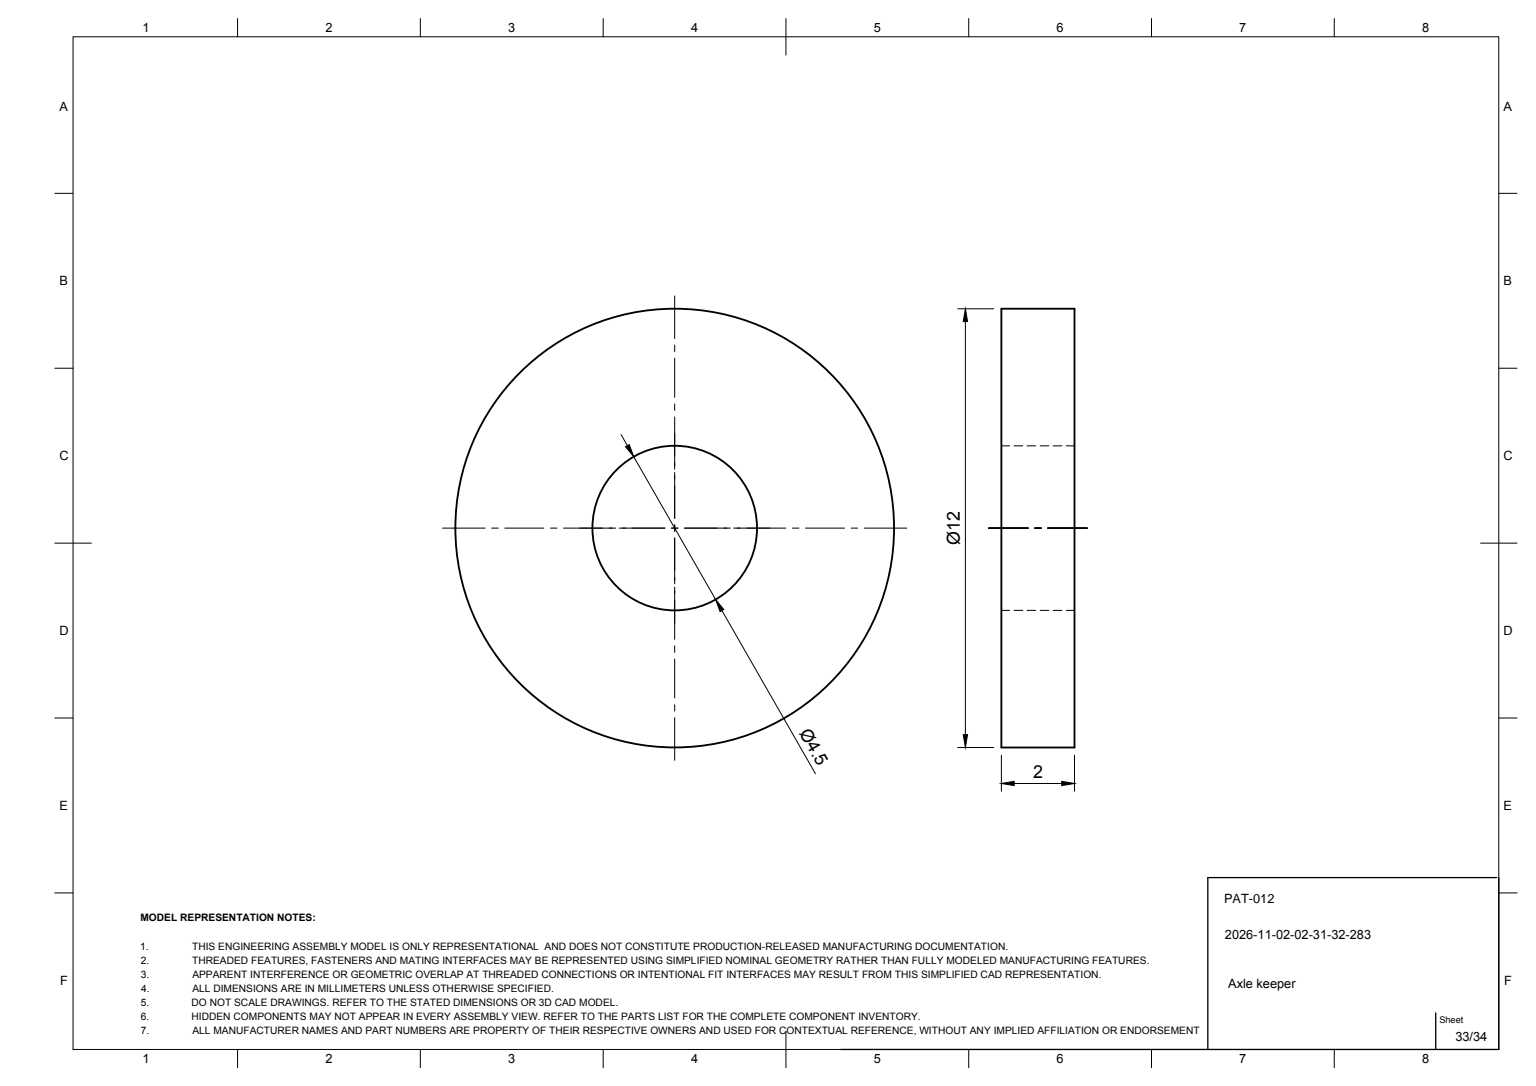
ISO-10303-21;
HEADER;
/* Generated by software containing ST-Developer
 * from STEP Tools, Inc. (www.steptools.com) 
 */

FILE_DESCRIPTION(
/* description */ ('Belt tensioner idler arm'),
/* implementation_level */ '2;1');

FILE_NAME(
/* name */ 'Axle keeper.step',
/* time_stamp */ '2026-10-28T03:22:15-07:00',
/* author */ (''),
/* organization */ (''),
/* preprocessor_version */ 'ST-DEVELOPER v20.2',
/* originating_system */ 'Autodesk Translation Framework v15.17.0.0',
/* authorisation */ '');

FILE_SCHEMA (('AUTOMOTIVE_DESIGN { 1 0 10303 214 3 1 1 }'));
ENDSEC;

DATA;
#10=MECHANICAL_DESIGN_GEOMETRIC_PRESENTATION_REPRESENTATION('',(#485),#12779);
#409=SHAPE_REPRESENTATION_RELATIONSHIP('SRR','None',#12958,#443);
#443=ADVANCED_BREP_SHAPE_REPRESENTATION('',(#524),#12775);
#485=STYLED_ITEM('',(#13184),#524);
#524=MANIFOLD_SOLID_BREP('Body1',#6222);
#648=FACE_BOUND('',#1611,.T.);
#649=FACE_BOUND('',#1613,.T.);
#810=PLANE('',#7218);
#811=PLANE('',#7219);
#1120=FACE_OUTER_BOUND('',#1608,.T.);
#1121=FACE_OUTER_BOUND('',#1609,.T.);
#1122=FACE_OUTER_BOUND('',#1610,.T.);
#1123=FACE_OUTER_BOUND('',#1612,.T.);
#1608=EDGE_LOOP('',(#5224,#5225,#5226,#5227));
#1609=EDGE_LOOP('',(#5228,#5229,#5230,#5231));
#1610=EDGE_LOOP('',(#5232));
#1611=EDGE_LOOP('',(#5233));
#1612=EDGE_LOOP('',(#5234));
#1613=EDGE_LOOP('',(#5235));
#1961=LINE('',#11940,#2310);
#1962=LINE('',#11946,#2311);
#2310=VECTOR('',#8911,0.225);
#2311=VECTOR('',#8918,0.6);
#2667=CIRCLE('',#7213,0.225);
#2668=CIRCLE('',#7214,0.225);
#2669=CIRCLE('',#7216,0.6);
#2670=CIRCLE('',#7217,0.6);
#3150=VERTEX_POINT('',#11937);
#3151=VERTEX_POINT('',#11939);
#3152=VERTEX_POINT('',#11943);
#3153=VERTEX_POINT('',#11945);
#3867=EDGE_CURVE('',#3150,#3150,#2667,.T.);
#3868=EDGE_CURVE('',#3150,#3151,#1961,.T.);
#3869=EDGE_CURVE('',#3151,#3151,#2668,.T.);
#3870=EDGE_CURVE('',#3152,#3152,#2669,.T.);
#3871=EDGE_CURVE('',#3152,#3153,#1962,.T.);
#3872=EDGE_CURVE('',#3153,#3153,#2670,.T.);
#5224=ORIENTED_EDGE('',*,*,#3867,.F.);
#5225=ORIENTED_EDGE('',*,*,#3868,.T.);
#5226=ORIENTED_EDGE('',*,*,#3869,.T.);
#5227=ORIENTED_EDGE('',*,*,#3868,.F.);
#5228=ORIENTED_EDGE('',*,*,#3870,.F.);
#5229=ORIENTED_EDGE('',*,*,#3871,.T.);
#5230=ORIENTED_EDGE('',*,*,#3872,.T.);
#5231=ORIENTED_EDGE('',*,*,#3871,.F.);
#5232=ORIENTED_EDGE('',*,*,#3870,.T.);
#5233=ORIENTED_EDGE('',*,*,#3867,.T.);
#5234=ORIENTED_EDGE('',*,*,#3872,.F.);
#5235=ORIENTED_EDGE('',*,*,#3869,.F.);
#5761=CYLINDRICAL_SURFACE('',#7212,0.225);
#5762=CYLINDRICAL_SURFACE('',#7215,0.6);
#6097=ADVANCED_FACE('',(#1120),#5761,.F.);
#6098=ADVANCED_FACE('',(#1121),#5762,.T.);
#6099=ADVANCED_FACE('',(#1122,#648),#810,.T.);
#6100=ADVANCED_FACE('',(#1123,#649),#811,.F.);
#6222=CLOSED_SHELL('',(#6097,#6098,#6099,#6100));
#7211=AXIS2_PLACEMENT_3D('',#11935,#8905,#8906);
#7212=AXIS2_PLACEMENT_3D('',#11936,#8907,#8908);
#7213=AXIS2_PLACEMENT_3D('',#11938,#8909,#8910);
#7214=AXIS2_PLACEMENT_3D('',#11941,#8912,#8913);
#7215=AXIS2_PLACEMENT_3D('',#11942,#8914,#8915);
#7216=AXIS2_PLACEMENT_3D('',#11944,#8916,#8917);
#7217=AXIS2_PLACEMENT_3D('',#11947,#8919,#8920);
#7218=AXIS2_PLACEMENT_3D('',#11948,#8921,#8922);
#7219=AXIS2_PLACEMENT_3D('',#11949,#8923,#8924);
#8905=DIRECTION('axis',(0.,0.,1.));
#8906=DIRECTION('refdir',(1.,0.,0.));
#8907=DIRECTION('center_axis',(0.,0.,1.));
#8908=DIRECTION('ref_axis',(1.,0.,0.));
#8909=DIRECTION('center_axis',(0.,0.,-1.));
#8910=DIRECTION('ref_axis',(1.,0.,0.));
#8911=DIRECTION('',(0.,0.,-1.));
#8912=DIRECTION('center_axis',(0.,0.,-1.));
#8913=DIRECTION('ref_axis',(1.,0.,0.));
#8914=DIRECTION('center_axis',(0.,0.,1.));
#8915=DIRECTION('ref_axis',(1.,0.,0.));
#8916=DIRECTION('center_axis',(0.,0.,1.));
#8917=DIRECTION('ref_axis',(1.,0.,0.));
#8918=DIRECTION('',(0.,0.,-1.));
#8919=DIRECTION('center_axis',(0.,0.,1.));
#8920=DIRECTION('ref_axis',(1.,0.,0.));
#8921=DIRECTION('center_axis',(0.,0.,1.));
#8922=DIRECTION('ref_axis',(1.,0.,0.));
#8923=DIRECTION('center_axis',(0.,0.,1.));
#8924=DIRECTION('ref_axis',(1.,0.,0.));
#11935=CARTESIAN_POINT('',(0.,0.,0.));
#11936=CARTESIAN_POINT('Origin',(9.,0.,9.));
#11937=CARTESIAN_POINT('',(8.775,-2.75545529808154E-17,9.2));
#11938=CARTESIAN_POINT('Origin',(9.,0.,9.2));
#11939=CARTESIAN_POINT('',(8.775,-2.75545529808154E-17,9.));
#11940=CARTESIAN_POINT('',(8.775,-2.75545529808154E-17,9.));
#11941=CARTESIAN_POINT('Origin',(9.,0.,9.));
#11942=CARTESIAN_POINT('Origin',(9.,0.,9.));
#11943=CARTESIAN_POINT('',(8.4,-7.34788079488412E-17,9.2));
#11944=CARTESIAN_POINT('Origin',(9.,0.,9.2));
#11945=CARTESIAN_POINT('',(8.4,-7.34788079488412E-17,9.));
#11946=CARTESIAN_POINT('',(8.4,-7.34788079488412E-17,9.));
#11947=CARTESIAN_POINT('Origin',(9.,0.,9.));
#11948=CARTESIAN_POINT('Origin',(9.,0.,9.2));
#11949=CARTESIAN_POINT('Origin',(9.,0.,9.));
#12735=UNCERTAINTY_MEASURE_WITH_UNIT(LENGTH_MEASURE(0.001),#12780,
'DISTANCE_ACCURACY_VALUE',
'Maximum model space distance between geometric entities at asserted c
onnectivities');
#12739=UNCERTAINTY_MEASURE_WITH_UNIT(LENGTH_MEASURE(0.001),#12780,
'DISTANCE_ACCURACY_VALUE',
'Maximum model space distance between geometric entities at asserted c
onnectivities');
#12775=(
GEOMETRIC_REPRESENTATION_CONTEXT(3)
GLOBAL_UNCERTAINTY_ASSIGNED_CONTEXT((#12735))
GLOBAL_UNIT_ASSIGNED_CONTEXT((#12780,#12782,#12783))
REPRESENTATION_CONTEXT('','3D')
);
#12779=(
GEOMETRIC_REPRESENTATION_CONTEXT(3)
GLOBAL_UNCERTAINTY_ASSIGNED_CONTEXT((#12739))
GLOBAL_UNIT_ASSIGNED_CONTEXT((#12780,#12782,#12783))
REPRESENTATION_CONTEXT('','3D')
);
#12780=(
LENGTH_UNIT()
NAMED_UNIT(*)
SI_UNIT(.CENTI.,.METRE.)
);
#12782=(
NAMED_UNIT(*)
PLANE_ANGLE_UNIT()
SI_UNIT($,.RADIAN.)
);
#12783=(
NAMED_UNIT(*)
SI_UNIT($,.STERADIAN.)
SOLID_ANGLE_UNIT()
);
#12819=SHAPE_DEFINITION_REPRESENTATION(#12887,#12958);
#12887=PRODUCT_DEFINITION_SHAPE('',$,#12998);
#12958=SHAPE_REPRESENTATION('',(#7211),#12775);
#12962=PRODUCT_DEFINITION_CONTEXT('part definition',#13081,'design');
#12998=PRODUCT_DEFINITION('Axle keeper','Axle keeper',#13037,#12962);
#13037=PRODUCT_DEFINITION_FORMATION('',$,#13118);
#13081=APPLICATION_CONTEXT(
'Core Data for Automotive Mechanical Design Process');
#13082=PRODUCT_CONTEXT('part definition',#13081,'mechanical');
#13118=PRODUCT('Axle keeper','Axle keeper','Axle keeper',(#13082));
#13178=COLOUR_RGB('Grey',0.48,0.52,0.57);
#13179=FILL_AREA_STYLE_COLOUR('',#13178);
#13180=FILL_AREA_STYLE('',(#13179));
#13181=SURFACE_STYLE_FILL_AREA(#13180);
#13182=SURFACE_SIDE_STYLE('',(#13181));
#13183=SURFACE_STYLE_USAGE(.BOTH.,#13182);
#13184=PRESENTATION_STYLE_ASSIGNMENT((#13183));
ENDSEC;
END-ISO-10303-21;
